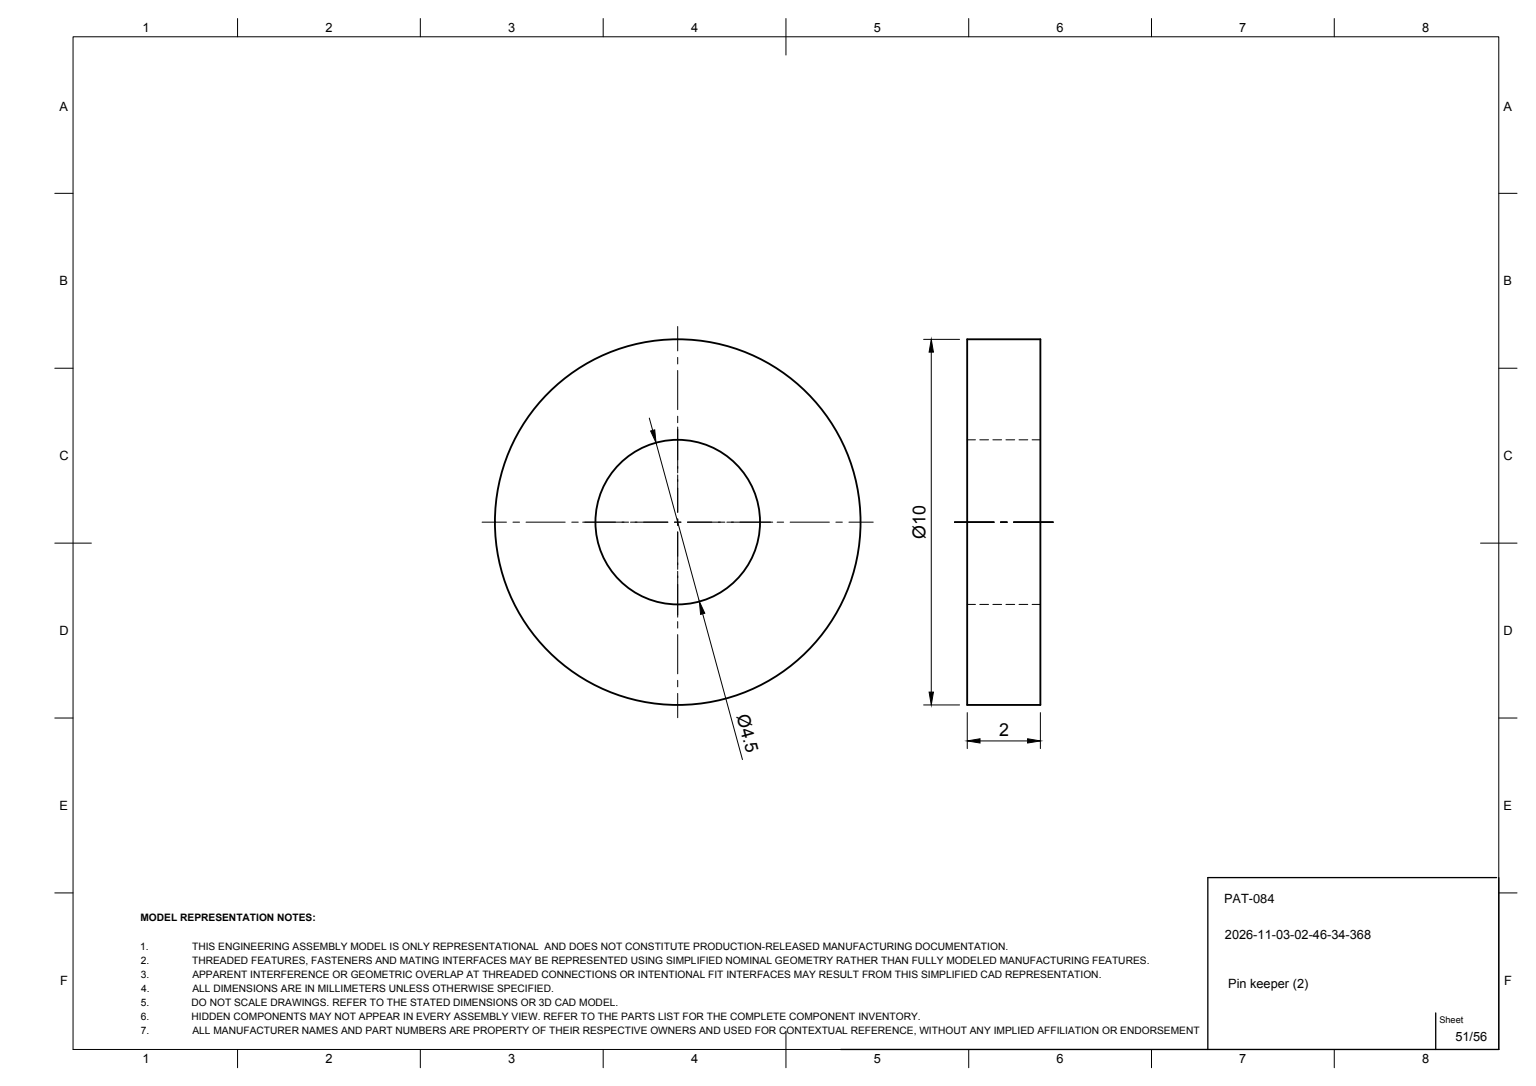
ISO-10303-21;
HEADER;
/* Generated by software containing ST-Developer
 * from STEP Tools, Inc. (www.steptools.com) 
 */

FILE_DESCRIPTION(
/* description */ ('Quick-return (Whitworth) mechanism'),
/* implementation_level */ '2;1');

FILE_NAME(
/* name */ 'Pin keeper (2).step',
/* time_stamp */ '2026-10-28T03:25:57-07:00',
/* author */ (''),
/* organization */ (''),
/* preprocessor_version */ 'ST-DEVELOPER v20.2',
/* originating_system */ 'Autodesk Translation Framework v15.17.0.0',
/* authorisation */ '');

FILE_SCHEMA (('AUTOMOTIVE_DESIGN { 1 0 10303 214 3 1 1 }'));
ENDSEC;

DATA;
#10=MECHANICAL_DESIGN_GEOMETRIC_PRESENTATION_REPRESENTATION('',(#536),#14878);
#440=SHAPE_REPRESENTATION_RELATIONSHIP('SRR','None',#15114,#484);
#484=ADVANCED_BREP_SHAPE_REPRESENTATION('',(#587),#14871);
#536=STYLED_ITEM('',(#15406),#587);
#587=MANIFOLD_SOLID_BREP('Body1',#7891);
#774=FACE_BOUND('',#2087,.T.);
#775=FACE_BOUND('',#2089,.T.);
#985=PLANE('',#9215);
#986=PLANE('',#9216);
#1435=FACE_OUTER_BOUND('',#2084,.T.);
#1436=FACE_OUTER_BOUND('',#2085,.T.);
#1437=FACE_OUTER_BOUND('',#2086,.T.);
#1438=FACE_OUTER_BOUND('',#2088,.T.);
#2084=EDGE_LOOP('',(#6838,#6839,#6840,#6841));
#2085=EDGE_LOOP('',(#6842,#6843,#6844,#6845));
#2086=EDGE_LOOP('',(#6846));
#2087=EDGE_LOOP('',(#6847));
#2088=EDGE_LOOP('',(#6848));
#2089=EDGE_LOOP('',(#6849));
#2541=LINE('',#14313,#3064);
#2542=LINE('',#14319,#3065);
#3064=VECTOR('',#11422,0.225);
#3065=VECTOR('',#11429,0.5);
#3597=CIRCLE('',#9210,0.225);
#3598=CIRCLE('',#9211,0.225);
#3599=CIRCLE('',#9213,0.5);
#3600=CIRCLE('',#9214,0.5);
#4166=VERTEX_POINT('',#14310);
#4167=VERTEX_POINT('',#14312);
#4168=VERTEX_POINT('',#14316);
#4169=VERTEX_POINT('',#14318);
#5076=EDGE_CURVE('',#4166,#4166,#3597,.T.);
#5077=EDGE_CURVE('',#4166,#4167,#2541,.T.);
#5078=EDGE_CURVE('',#4167,#4167,#3598,.T.);
#5079=EDGE_CURVE('',#4168,#4168,#3599,.T.);
#5080=EDGE_CURVE('',#4168,#4169,#2542,.T.);
#5081=EDGE_CURVE('',#4169,#4169,#3600,.T.);
#6838=ORIENTED_EDGE('',*,*,#5076,.F.);
#6839=ORIENTED_EDGE('',*,*,#5077,.T.);
#6840=ORIENTED_EDGE('',*,*,#5078,.T.);
#6841=ORIENTED_EDGE('',*,*,#5077,.F.);
#6842=ORIENTED_EDGE('',*,*,#5079,.F.);
#6843=ORIENTED_EDGE('',*,*,#5080,.T.);
#6844=ORIENTED_EDGE('',*,*,#5081,.T.);
#6845=ORIENTED_EDGE('',*,*,#5080,.F.);
#6846=ORIENTED_EDGE('',*,*,#5079,.T.);
#6847=ORIENTED_EDGE('',*,*,#5076,.T.);
#6848=ORIENTED_EDGE('',*,*,#5081,.F.);
#6849=ORIENTED_EDGE('',*,*,#5078,.F.);
#7368=CYLINDRICAL_SURFACE('',#9209,0.225);
#7369=CYLINDRICAL_SURFACE('',#9212,0.5);
#7766=ADVANCED_FACE('',(#1435),#7368,.F.);
#7767=ADVANCED_FACE('',(#1436),#7369,.T.);
#7768=ADVANCED_FACE('',(#1437,#774),#985,.T.);
#7769=ADVANCED_FACE('',(#1438,#775),#986,.F.);
#7891=CLOSED_SHELL('',(#7766,#7767,#7768,#7769));
#9208=AXIS2_PLACEMENT_3D('',#14308,#11416,#11417);
#9209=AXIS2_PLACEMENT_3D('',#14309,#11418,#11419);
#9210=AXIS2_PLACEMENT_3D('',#14311,#11420,#11421);
#9211=AXIS2_PLACEMENT_3D('',#14314,#11423,#11424);
#9212=AXIS2_PLACEMENT_3D('',#14315,#11425,#11426);
#9213=AXIS2_PLACEMENT_3D('',#14317,#11427,#11428);
#9214=AXIS2_PLACEMENT_3D('',#14320,#11430,#11431);
#9215=AXIS2_PLACEMENT_3D('',#14321,#11432,#11433);
#9216=AXIS2_PLACEMENT_3D('',#14322,#11434,#11435);
#11416=DIRECTION('axis',(0.,0.,1.));
#11417=DIRECTION('refdir',(1.,0.,0.));
#11418=DIRECTION('center_axis',(0.,0.,1.));
#11419=DIRECTION('ref_axis',(1.,0.,0.));
#11420=DIRECTION('center_axis',(0.,0.,-1.));
#11421=DIRECTION('ref_axis',(1.,0.,0.));
#11422=DIRECTION('',(0.,0.,-1.));
#11423=DIRECTION('center_axis',(0.,0.,-1.));
#11424=DIRECTION('ref_axis',(1.,0.,0.));
#11425=DIRECTION('center_axis',(0.,0.,1.));
#11426=DIRECTION('ref_axis',(1.,0.,0.));
#11427=DIRECTION('center_axis',(0.,0.,1.));
#11428=DIRECTION('ref_axis',(1.,0.,0.));
#11429=DIRECTION('',(0.,0.,-1.));
#11430=DIRECTION('center_axis',(0.,0.,1.));
#11431=DIRECTION('ref_axis',(1.,0.,0.));
#11432=DIRECTION('center_axis',(0.,0.,1.));
#11433=DIRECTION('ref_axis',(1.,0.,0.));
#11434=DIRECTION('center_axis',(0.,0.,1.));
#11435=DIRECTION('ref_axis',(1.,0.,0.));
#14308=CARTESIAN_POINT('',(0.,0.,0.));
#14309=CARTESIAN_POINT('Origin',(9.16515138991168,16.,9.8));
#14310=CARTESIAN_POINT('',(8.94015138991168,16.,10.));
#14311=CARTESIAN_POINT('Origin',(9.16515138991168,16.,10.));
#14312=CARTESIAN_POINT('',(8.94015138991168,16.,9.8));
#14313=CARTESIAN_POINT('',(8.94015138991168,16.,9.8));
#14314=CARTESIAN_POINT('Origin',(9.16515138991168,16.,9.8));
#14315=CARTESIAN_POINT('Origin',(9.16515138991168,16.,9.8));
#14316=CARTESIAN_POINT('',(8.66515138991168,16.,10.));
#14317=CARTESIAN_POINT('Origin',(9.16515138991168,16.,10.));
#14318=CARTESIAN_POINT('',(8.66515138991168,16.,9.8));
#14319=CARTESIAN_POINT('',(8.66515138991168,16.,9.8));
#14320=CARTESIAN_POINT('Origin',(9.16515138991168,16.,9.8));
#14321=CARTESIAN_POINT('Origin',(9.16515138991168,16.,10.));
#14322=CARTESIAN_POINT('Origin',(9.16515138991168,16.,9.8));
#14817=UNCERTAINTY_MEASURE_WITH_UNIT(LENGTH_MEASURE(0.001),#14879,
'DISTANCE_ACCURACY_VALUE',
'Maximum model space distance between geometric entities at asserted c
onnectivities');
#14824=UNCERTAINTY_MEASURE_WITH_UNIT(LENGTH_MEASURE(0.001),#14879,
'DISTANCE_ACCURACY_VALUE',
'Maximum model space distance between geometric entities at asserted c
onnectivities');
#14871=(
GEOMETRIC_REPRESENTATION_CONTEXT(3)
GLOBAL_UNCERTAINTY_ASSIGNED_CONTEXT((#14817))
GLOBAL_UNIT_ASSIGNED_CONTEXT((#14879,#14881,#14882))
REPRESENTATION_CONTEXT('','3D')
);
#14878=(
GEOMETRIC_REPRESENTATION_CONTEXT(3)
GLOBAL_UNCERTAINTY_ASSIGNED_CONTEXT((#14824))
GLOBAL_UNIT_ASSIGNED_CONTEXT((#14879,#14881,#14882))
REPRESENTATION_CONTEXT('','3D')
);
#14879=(
LENGTH_UNIT()
NAMED_UNIT(*)
SI_UNIT(.CENTI.,.METRE.)
);
#14881=(
NAMED_UNIT(*)
PLANE_ANGLE_UNIT()
SI_UNIT($,.RADIAN.)
);
#14882=(
NAMED_UNIT(*)
SI_UNIT($,.STERADIAN.)
SOLID_ANGLE_UNIT()
);
#14929=SHAPE_DEFINITION_REPRESENTATION(#14991,#15114);
#14991=PRODUCT_DEFINITION_SHAPE('',$,#15168);
#15114=SHAPE_REPRESENTATION('',(#9208),#14871);
#15121=PRODUCT_DEFINITION_CONTEXT('part definition',#15282,'design');
#15168=PRODUCT_DEFINITION('Pin keeper (2)','Pin keeper (2)',#15221,#15121);
#15221=PRODUCT_DEFINITION_FORMATION('',$,#15330);
#15282=APPLICATION_CONTEXT(
'Core Data for Automotive Mechanical Design Process');
#15283=PRODUCT_CONTEXT('part definition',#15282,'mechanical');
#15330=PRODUCT('Pin keeper (2)','Pin keeper (2)','Pin keeper (2)',(#15283));
#15400=COLOUR_RGB('Grey',0.48,0.52,0.57);
#15401=FILL_AREA_STYLE_COLOUR('',#15400);
#15402=FILL_AREA_STYLE('',(#15401));
#15403=SURFACE_STYLE_FILL_AREA(#15402);
#15404=SURFACE_SIDE_STYLE('',(#15403));
#15405=SURFACE_STYLE_USAGE(.BOTH.,#15404);
#15406=PRESENTATION_STYLE_ASSIGNMENT((#15405));
ENDSEC;
END-ISO-10303-21;
